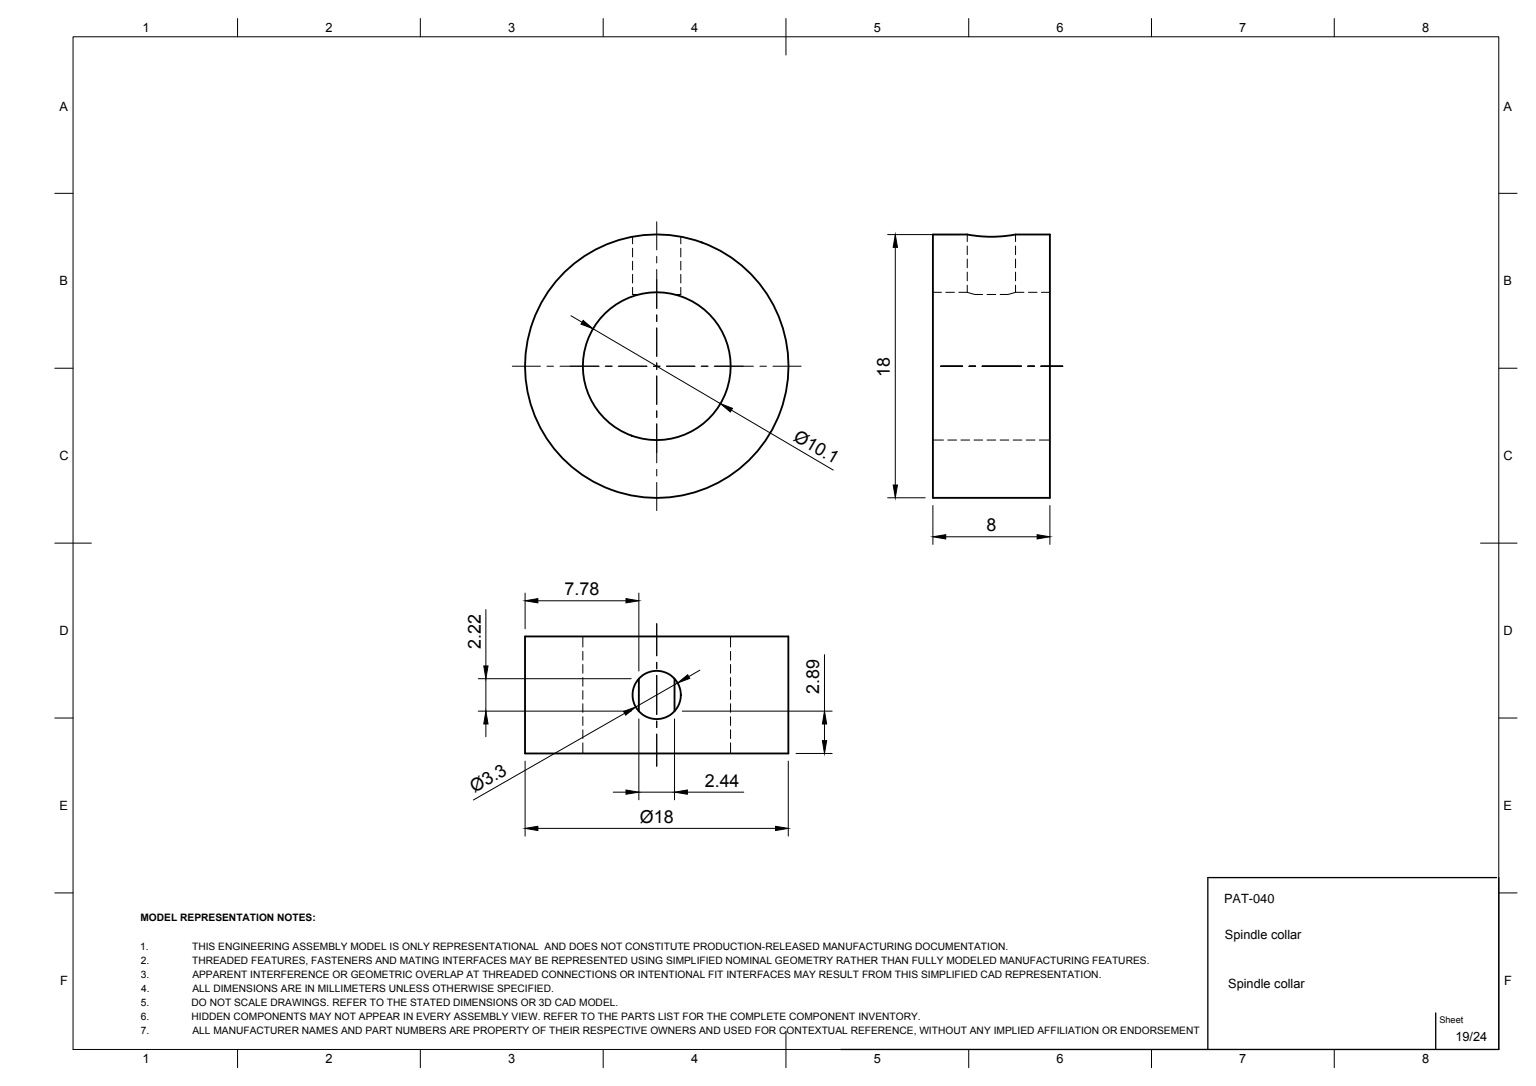
ISO-10303-21;
HEADER;
/* Generated by software containing ST-Developer
 * from STEP Tools, Inc. (www.steptools.com) 
 */

FILE_DESCRIPTION(
/* description */ ('Four-bar tabletop demonstrator'),
/* implementation_level */ '2;1');

FILE_NAME(
/* name */ 'Spindle collar.step',
/* time_stamp */ '2026-10-29T17:05:23-07:00',
/* author */ (''),
/* organization */ (''),
/* preprocessor_version */ 'ST-DEVELOPER v20.2',
/* originating_system */ 'Autodesk Translation Framework v15.17.0.0',
/* authorisation */ '');

FILE_SCHEMA (('AUTOMOTIVE_DESIGN { 1 0 10303 214 3 1 1 }'));
ENDSEC;

DATA;
#10=MECHANICAL_DESIGN_GEOMETRIC_PRESENTATION_REPRESENTATION('',(#358),#6705);
#302=B_SPLINE_CURVE_WITH_KNOTS('',3,(#6493,#6494,#6495,#6496,#6497,#6498,
#6499,#6500,#6501,#6502,#6503,#6504,#6505,#6506),.UNSPECIFIED.,.F.,.F.,
(4,2,2,2,2,2,4),(0.618551524396293,0.626563103102765,0.689203386094988,
0.751843669087211,0.814483952079434,0.877124235071657,0.88513581377813),
 .UNSPECIFIED.);
#303=B_SPLINE_CURVE_WITH_KNOTS('',3,(#6510,#6511,#6512,#6513,#6514,#6515,
#6516,#6517),.UNSPECIFIED.,.F.,.F.,(4,2,2,4),(0.250614556362404,0.313254839354627,
0.37589512234685,0.383906701053323),.UNSPECIFIED.);
#304=B_SPLINE_CURVE_WITH_KNOTS('',3,(#6521,#6522,#6523,#6524,#6525,#6526,
#6527,#6528,#6529,#6530,#6531,#6532,#6533,#6534,#6535,#6536,#6537,#6538,
#6539,#6540,#6541,#6542,#6543,#6544,#6545,#6546),.UNSPECIFIED.,.F.,.F.,
(4,2,2,2,2,2,2,2,2,2,2,2,4),(0.,0.0623062782223143,0.124612556444629,0.186916384615149,
0.249220212785669,0.31152404095619,0.37382786912671,0.436134147349024,0.498440425571339,
0.560746703793653,0.623052982015967,0.685356810186488,0.747660638357008),
 .UNSPECIFIED.);
#305=B_SPLINE_CURVE_WITH_KNOTS('',3,(#6547,#6548,#6549,#6550,#6551,#6552,
#6553,#6554,#6555,#6556),.UNSPECIFIED.,.F.,.F.,(4,2,2,2,4),(0.747660638357008,
0.809964466527528,0.872268294698049,0.934574572920363,0.996880851142677),
 .UNSPECIFIED.);
#306=B_SPLINE_CURVE_WITH_KNOTS('',3,(#6557,#6558,#6559,#6560,#6561,#6562,
#6563,#6564),.UNSPECIFIED.,.F.,.F.,(4,2,2,4),(0.117322411671485,0.125333990377958,
0.187974273370181,0.250614556362404),.UNSPECIFIED.);
#320=SHAPE_REPRESENTATION_RELATIONSHIP('SRR','None',#6830,#335);
#335=ADVANCED_BREP_SHAPE_REPRESENTATION('',(#379),#6703);
#358=STYLED_ITEM('',(#6982),#379);
#379=MANIFOLD_SOLID_BREP('Body1',#3404);
#457=FACE_BOUND('',#1030,.T.);
#458=FACE_BOUND('',#1032,.T.);
#459=FACE_BOUND('',#1034,.T.);
#460=FACE_BOUND('',#1036,.T.);
#549=PLANE('',#4007);
#550=PLANE('',#4011);
#551=PLANE('',#4018);
#552=PLANE('',#4019);
#747=FACE_OUTER_BOUND('',#1026,.T.);
#748=FACE_OUTER_BOUND('',#1027,.T.);
#749=FACE_OUTER_BOUND('',#1028,.T.);
#750=FACE_OUTER_BOUND('',#1029,.T.);
#751=FACE_OUTER_BOUND('',#1031,.T.);
#752=FACE_OUTER_BOUND('',#1033,.T.);
#753=FACE_OUTER_BOUND('',#1035,.T.);
#1026=EDGE_LOOP('',(#3026,#3027));
#1027=EDGE_LOOP('',(#3028,#3029,#3030,#3031,#3032,#3033,#3034,#3035,#3036));
#1028=EDGE_LOOP('',(#3037,#3038));
#1029=EDGE_LOOP('',(#3039,#3040,#3041,#3042));
#1030=EDGE_LOOP('',(#3043,#3044,#3045,#3046,#3047));
#1031=EDGE_LOOP('',(#3048,#3049,#3050,#3051));
#1032=EDGE_LOOP('',(#3052,#3053));
#1033=EDGE_LOOP('',(#3054));
#1034=EDGE_LOOP('',(#3055));
#1035=EDGE_LOOP('',(#3056));
#1036=EDGE_LOOP('',(#3057));
#1194=LINE('',#6489,#1364);
#1195=LINE('',#6519,#1365);
#1196=LINE('',#6566,#1366);
#1197=LINE('',#6571,#1367);
#1198=LINE('',#6577,#1368);
#1364=VECTOR('',#5083,1.);
#1365=VECTOR('',#5090,0.165);
#1366=VECTOR('',#5093,1.);
#1367=VECTOR('',#5098,0.505);
#1368=VECTOR('',#5105,0.9);
#1591=CIRCLE('',#4008,0.165);
#1592=CIRCLE('',#4010,0.165);
#1593=CIRCLE('',#4013,0.505);
#1594=CIRCLE('',#4014,0.505);
#1595=CIRCLE('',#4016,0.9);
#1596=CIRCLE('',#4017,0.9);
#1854=VERTEX_POINT('',#6487);
#1855=VERTEX_POINT('',#6488);
#1856=VERTEX_POINT('',#6492);
#1857=VERTEX_POINT('',#6507);
#1858=VERTEX_POINT('',#6509);
#1859=VERTEX_POINT('',#6518);
#1860=VERTEX_POINT('',#6520);
#1861=VERTEX_POINT('',#6568);
#1862=VERTEX_POINT('',#6570);
#1863=VERTEX_POINT('',#6574);
#1864=VERTEX_POINT('',#6576);
#2249=EDGE_CURVE('',#1854,#1855,#1194,.T.);
#2250=EDGE_CURVE('',#1854,#1855,#1591,.T.);
#2251=EDGE_CURVE('',#1856,#1854,#302,.T.);
#2252=EDGE_CURVE('',#1857,#1856,#1592,.T.);
#2253=EDGE_CURVE('',#1858,#1857,#303,.T.);
#2254=EDGE_CURVE('',#1858,#1859,#1195,.T.);
#2255=EDGE_CURVE('',#1860,#1859,#304,.T.);
#2256=EDGE_CURVE('',#1859,#1860,#305,.T.);
#2257=EDGE_CURVE('',#1855,#1858,#306,.T.);
#2258=EDGE_CURVE('',#1857,#1856,#1196,.T.);
#2259=EDGE_CURVE('',#1861,#1861,#1593,.T.);
#2260=EDGE_CURVE('',#1861,#1862,#1197,.T.);
#2261=EDGE_CURVE('',#1862,#1862,#1594,.T.);
#2262=EDGE_CURVE('',#1863,#1863,#1595,.T.);
#2263=EDGE_CURVE('',#1863,#1864,#1198,.T.);
#2264=EDGE_CURVE('',#1864,#1864,#1596,.T.);
#3026=ORIENTED_EDGE('',*,*,#2249,.F.);
#3027=ORIENTED_EDGE('',*,*,#2250,.T.);
#3028=ORIENTED_EDGE('',*,*,#2251,.F.);
#3029=ORIENTED_EDGE('',*,*,#2252,.F.);
#3030=ORIENTED_EDGE('',*,*,#2253,.F.);
#3031=ORIENTED_EDGE('',*,*,#2254,.T.);
#3032=ORIENTED_EDGE('',*,*,#2255,.F.);
#3033=ORIENTED_EDGE('',*,*,#2256,.F.);
#3034=ORIENTED_EDGE('',*,*,#2254,.F.);
#3035=ORIENTED_EDGE('',*,*,#2257,.F.);
#3036=ORIENTED_EDGE('',*,*,#2250,.F.);
#3037=ORIENTED_EDGE('',*,*,#2258,.F.);
#3038=ORIENTED_EDGE('',*,*,#2252,.T.);
#3039=ORIENTED_EDGE('',*,*,#2259,.F.);
#3040=ORIENTED_EDGE('',*,*,#2260,.T.);
#3041=ORIENTED_EDGE('',*,*,#2261,.T.);
#3042=ORIENTED_EDGE('',*,*,#2260,.F.);
#3043=ORIENTED_EDGE('',*,*,#2257,.T.);
#3044=ORIENTED_EDGE('',*,*,#2253,.T.);
#3045=ORIENTED_EDGE('',*,*,#2258,.T.);
#3046=ORIENTED_EDGE('',*,*,#2251,.T.);
#3047=ORIENTED_EDGE('',*,*,#2249,.T.);
#3048=ORIENTED_EDGE('',*,*,#2262,.F.);
#3049=ORIENTED_EDGE('',*,*,#2263,.T.);
#3050=ORIENTED_EDGE('',*,*,#2264,.T.);
#3051=ORIENTED_EDGE('',*,*,#2263,.F.);
#3052=ORIENTED_EDGE('',*,*,#2255,.T.);
#3053=ORIENTED_EDGE('',*,*,#2256,.T.);
#3054=ORIENTED_EDGE('',*,*,#2262,.T.);
#3055=ORIENTED_EDGE('',*,*,#2259,.T.);
#3056=ORIENTED_EDGE('',*,*,#2264,.F.);
#3057=ORIENTED_EDGE('',*,*,#2261,.F.);
#3174=CYLINDRICAL_SURFACE('',#4009,0.165);
#3175=CYLINDRICAL_SURFACE('',#4012,0.505);
#3176=CYLINDRICAL_SURFACE('',#4015,0.9);
#3363=ADVANCED_FACE('',(#747),#549,.T.);
#3364=ADVANCED_FACE('',(#748),#3174,.F.);
#3365=ADVANCED_FACE('',(#749),#550,.T.);
#3366=ADVANCED_FACE('',(#750,#457),#3175,.F.);
#3367=ADVANCED_FACE('',(#751,#458),#3176,.T.);
#3368=ADVANCED_FACE('',(#752,#459),#551,.T.);
#3369=ADVANCED_FACE('',(#753,#460),#552,.F.);
#3404=CLOSED_SHELL('',(#3363,#3364,#3365,#3366,#3367,#3368,#3369));
#4006=AXIS2_PLACEMENT_3D('',#6485,#5079,#5080);
#4007=AXIS2_PLACEMENT_3D('',#6486,#5081,#5082);
#4008=AXIS2_PLACEMENT_3D('',#6490,#5084,#5085);
#4009=AXIS2_PLACEMENT_3D('',#6491,#5086,#5087);
#4010=AXIS2_PLACEMENT_3D('',#6508,#5088,#5089);
#4011=AXIS2_PLACEMENT_3D('',#6565,#5091,#5092);
#4012=AXIS2_PLACEMENT_3D('',#6567,#5094,#5095);
#4013=AXIS2_PLACEMENT_3D('',#6569,#5096,#5097);
#4014=AXIS2_PLACEMENT_3D('',#6572,#5099,#5100);
#4015=AXIS2_PLACEMENT_3D('',#6573,#5101,#5102);
#4016=AXIS2_PLACEMENT_3D('',#6575,#5103,#5104);
#4017=AXIS2_PLACEMENT_3D('',#6578,#5106,#5107);
#4018=AXIS2_PLACEMENT_3D('',#6579,#5108,#5109);
#4019=AXIS2_PLACEMENT_3D('',#6580,#5110,#5111);
#5079=DIRECTION('axis',(0.,0.,1.));
#5080=DIRECTION('refdir',(1.,0.,0.));
#5081=DIRECTION('center_axis',(1.,0.,0.));
#5082=DIRECTION('ref_axis',(0.,0.,-1.));
#5083=DIRECTION('',(0.,0.,1.));
#5084=DIRECTION('center_axis',(1.,0.,0.));
#5085=DIRECTION('ref_axis',(0.,0.,-1.));
#5086=DIRECTION('center_axis',(1.,0.,0.));
#5087=DIRECTION('ref_axis',(0.,0.,-1.));
#5088=DIRECTION('center_axis',(1.,0.,0.));
#5089=DIRECTION('ref_axis',(0.,0.,-1.));
#5090=DIRECTION('',(1.,0.,0.));
#5091=DIRECTION('center_axis',(1.,0.,0.));
#5092=DIRECTION('ref_axis',(0.,0.,-1.));
#5093=DIRECTION('',(0.,0.,-1.));
#5094=DIRECTION('center_axis',(0.,0.,1.));
#5095=DIRECTION('ref_axis',(1.,0.,0.));
#5096=DIRECTION('center_axis',(0.,0.,-1.));
#5097=DIRECTION('ref_axis',(1.,0.,0.));
#5098=DIRECTION('',(0.,0.,-1.));
#5099=DIRECTION('center_axis',(0.,0.,-1.));
#5100=DIRECTION('ref_axis',(1.,0.,0.));
#5101=DIRECTION('center_axis',(0.,0.,1.));
#5102=DIRECTION('ref_axis',(1.,0.,0.));
#5103=DIRECTION('center_axis',(0.,0.,1.));
#5104=DIRECTION('ref_axis',(1.,0.,0.));
#5105=DIRECTION('',(0.,0.,-1.));
#5106=DIRECTION('center_axis',(0.,0.,1.));
#5107=DIRECTION('ref_axis',(1.,0.,0.));
#5108=DIRECTION('center_axis',(0.,0.,1.));
#5109=DIRECTION('ref_axis',(1.,0.,0.));
#5110=DIRECTION('center_axis',(0.,0.,1.));
#5111=DIRECTION('ref_axis',(1.,0.,0.));
#6485=CARTESIAN_POINT('',(0.,0.,0.));
#6486=CARTESIAN_POINT('Origin',(0.49,0.,1.4));
#6487=CARTESIAN_POINT('',(0.49,0.122167917228706,1.28909463493591));
#6488=CARTESIAN_POINT('',(0.49,0.122167917228706,1.51090536506409));
#6489=CARTESIAN_POINT('',(0.49,0.122167917228706,1.));
#6490=CARTESIAN_POINT('Origin',(0.49,0.,1.4));
#6491=CARTESIAN_POINT('Origin',(0.49,0.,1.4));
#6492=CARTESIAN_POINT('',(0.49,-0.122167917228706,1.28909463493591));
#6493=CARTESIAN_POINT('Ctrl Pts',(0.49,-0.122167917228706,1.28909463493591));
#6494=CARTESIAN_POINT('Ctrl Pts',(0.490448531679987,-0.120368913626296,
1.28711294069536));
#6495=CARTESIAN_POINT('Ctrl Pts',(0.490895245371685,-0.118534896565231,
1.28518965877367));
#6496=CARTESIAN_POINT('Ctrl Pts',(0.494795015531646,-0.102111993019358,
1.2687667552278));
#6497=CARTESIAN_POINT('Ctrl Pts',(0.498442514607594,-0.0836597150224318,
1.25609154388858));
#6498=CARTESIAN_POINT('Ctrl Pts',(0.50357781976106,-0.0430495960471595,
1.23920409039234));
#6499=CARTESIAN_POINT('Ctrl Pts',(0.505,-0.020880094330741,1.235));
#6500=CARTESIAN_POINT('Ctrl Pts',(0.505,0.020880094330741,1.235));
#6501=CARTESIAN_POINT('Ctrl Pts',(0.50357781976106,0.0430495960471595,1.23920409039234));
#6502=CARTESIAN_POINT('Ctrl Pts',(0.498442514607594,0.0836597150224318,
1.25609154388858));
#6503=CARTESIAN_POINT('Ctrl Pts',(0.494795015531646,0.102111993019358,1.2687667552278));
#6504=CARTESIAN_POINT('Ctrl Pts',(0.490895245371684,0.118534896565231,1.28518965877367));
#6505=CARTESIAN_POINT('Ctrl Pts',(0.490448531679987,0.120368913626296,1.28711294069536));
#6506=CARTESIAN_POINT('Ctrl Pts',(0.49,0.122167917228706,1.28909463493591));
#6507=CARTESIAN_POINT('',(0.49,-0.122167917228706,1.51090536506409));
#6508=CARTESIAN_POINT('Origin',(0.49,0.,1.4));
#6509=CARTESIAN_POINT('',(0.505,-1.70422299968729E-17,1.565));
#6510=CARTESIAN_POINT('Ctrl Pts',(0.505,-6.93889390390723E-18,1.565));
#6511=CARTESIAN_POINT('Ctrl Pts',(0.505,-0.020880094330741,1.565));
#6512=CARTESIAN_POINT('Ctrl Pts',(0.50357781976106,-0.0430495960471595,
1.56079590960766));
#6513=CARTESIAN_POINT('Ctrl Pts',(0.498442514607594,-0.0836597150224318,
1.54390845611142));
#6514=CARTESIAN_POINT('Ctrl Pts',(0.494795015531646,-0.102111993019358,
1.5312332447722));
#6515=CARTESIAN_POINT('Ctrl Pts',(0.490895245371684,-0.118534896565231,
1.51481034122633));
#6516=CARTESIAN_POINT('Ctrl Pts',(0.490448531679987,-0.120368913626296,
1.51288705930464));
#6517=CARTESIAN_POINT('Ctrl Pts',(0.49,-0.122167917228706,1.51090536506409));
#6518=CARTESIAN_POINT('',(0.9,-2.02066721859313E-17,1.565));
#6519=CARTESIAN_POINT('',(0.49,-2.02066721859313E-17,1.565));
#6520=CARTESIAN_POINT('',(0.884745726183518,0.165,1.4));
#6521=CARTESIAN_POINT('Ctrl Pts',(0.884745726183518,0.165,1.4));
#6522=CARTESIAN_POINT('Ctrl Pts',(0.884745726183518,0.165,1.37923124059256));
#6523=CARTESIAN_POINT('Ctrl Pts',(0.885552759505264,0.160839719007584,1.35711110492666));
#6524=CARTESIAN_POINT('Ctrl Pts',(0.888448648150043,0.143986470216691,1.31647293736623));
#6525=CARTESIAN_POINT('Ctrl Pts',(0.890493604851638,0.131295993814186,1.29795075602263));
#6526=CARTESIAN_POINT('Ctrl Pts',(0.89431723432394,0.102049819008125,1.26870458121656));
#6527=CARTESIAN_POINT('Ctrl Pts',(0.896347088899543,0.0835273920906824,
1.25601365401642));
#6528=CARTESIAN_POINT('Ctrl Pts',(0.899208271860583,0.0428883760934127,
1.23916007816136));
#6529=CARTESIAN_POINT('Ctrl Pts',(0.9,0.0207679427235068,1.235));
#6530=CARTESIAN_POINT('Ctrl Pts',(0.9,-0.0207679427235068,1.235));
#6531=CARTESIAN_POINT('Ctrl Pts',(0.899208271860583,-0.0428883760934127,
1.23916007816136));
#6532=CARTESIAN_POINT('Ctrl Pts',(0.896347088899543,-0.0835273920906823,
1.25601365401642));
#6533=CARTESIAN_POINT('Ctrl Pts',(0.89431723432394,-0.102049819008125,1.26870458121656));
#6534=CARTESIAN_POINT('Ctrl Pts',(0.890493604851638,-0.131295993814186,
1.29795075602263));
#6535=CARTESIAN_POINT('Ctrl Pts',(0.888448648150043,-0.143986470216691,
1.31647293736623));
#6536=CARTESIAN_POINT('Ctrl Pts',(0.885552759505264,-0.160839719007584,
1.35711110492666));
#6537=CARTESIAN_POINT('Ctrl Pts',(0.884745726183518,-0.165,1.37923124059256));
#6538=CARTESIAN_POINT('Ctrl Pts',(0.884745726183518,-0.165,1.42076875940744));
#6539=CARTESIAN_POINT('Ctrl Pts',(0.885552759505264,-0.160839719007584,
1.44288889507334));
#6540=CARTESIAN_POINT('Ctrl Pts',(0.888448648150043,-0.14398647021669,1.48352706263377));
#6541=CARTESIAN_POINT('Ctrl Pts',(0.890493604851638,-0.131295993814186,
1.50204924397737));
#6542=CARTESIAN_POINT('Ctrl Pts',(0.89431723432394,-0.102049819008125,1.53129541878344));
#6543=CARTESIAN_POINT('Ctrl Pts',(0.896347088899543,-0.0835273920906824,
1.54398634598358));
#6544=CARTESIAN_POINT('Ctrl Pts',(0.899208271860583,-0.0428883760934128,
1.56083992183864));
#6545=CARTESIAN_POINT('Ctrl Pts',(0.9,-0.0207679427235068,1.565));
#6546=CARTESIAN_POINT('Ctrl Pts',(0.9,-6.93889390390723E-18,1.565));
#6547=CARTESIAN_POINT('Ctrl Pts',(0.9,-3.46944695195361E-17,1.565));
#6548=CARTESIAN_POINT('Ctrl Pts',(0.9,0.0207679427235068,1.565));
#6549=CARTESIAN_POINT('Ctrl Pts',(0.899208271860583,0.0428883760934127,
1.56083992183864));
#6550=CARTESIAN_POINT('Ctrl Pts',(0.896347088899543,0.0835273920906824,
1.54398634598358));
#6551=CARTESIAN_POINT('Ctrl Pts',(0.89431723432394,0.102049819008125,1.53129541878344));
#6552=CARTESIAN_POINT('Ctrl Pts',(0.890493604851638,0.131295993814186,1.50204924397737));
#6553=CARTESIAN_POINT('Ctrl Pts',(0.888448648150043,0.143986470216691,1.48352706263377));
#6554=CARTESIAN_POINT('Ctrl Pts',(0.885552759505264,0.160839719007584,1.44288889507334));
#6555=CARTESIAN_POINT('Ctrl Pts',(0.884745726183518,0.165,1.42076875940744));
#6556=CARTESIAN_POINT('Ctrl Pts',(0.884745726183518,0.165,1.4));
#6557=CARTESIAN_POINT('Ctrl Pts',(0.49,0.122167917228706,1.51090536506409));
#6558=CARTESIAN_POINT('Ctrl Pts',(0.490448531679987,0.120368913626296,1.51288705930464));
#6559=CARTESIAN_POINT('Ctrl Pts',(0.490895245371685,0.118534896565231,1.51481034122633));
#6560=CARTESIAN_POINT('Ctrl Pts',(0.494795015531646,0.102111993019358,1.5312332447722));
#6561=CARTESIAN_POINT('Ctrl Pts',(0.498442514607594,0.0836597150224318,
1.54390845611142));
#6562=CARTESIAN_POINT('Ctrl Pts',(0.50357781976106,0.0430495960471594,1.56079590960766));
#6563=CARTESIAN_POINT('Ctrl Pts',(0.505,0.020880094330741,1.565));
#6564=CARTESIAN_POINT('Ctrl Pts',(0.505,0.,1.565));
#6565=CARTESIAN_POINT('Origin',(0.49,0.,1.4));
#6566=CARTESIAN_POINT('',(0.49,-0.122167917228706,1.));
#6567=CARTESIAN_POINT('Origin',(0.,0.,1.));
#6568=CARTESIAN_POINT('',(-0.505,-6.18446633569413E-17,1.8));
#6569=CARTESIAN_POINT('Origin',(0.,0.,1.8));
#6570=CARTESIAN_POINT('',(-0.505,-6.18446633569413E-17,1.));
#6571=CARTESIAN_POINT('',(-0.505,-6.18446633569413E-17,1.));
#6572=CARTESIAN_POINT('Origin',(0.,0.,1.));
#6573=CARTESIAN_POINT('Origin',(0.,0.,1.));
#6574=CARTESIAN_POINT('',(-0.9,-1.10218211923262E-16,1.8));
#6575=CARTESIAN_POINT('Origin',(0.,0.,1.8));
#6576=CARTESIAN_POINT('',(-0.9,-1.10218211923262E-16,1.));
#6577=CARTESIAN_POINT('',(-0.9,-1.10218211923262E-16,1.));
#6578=CARTESIAN_POINT('Origin',(0.,0.,1.));
#6579=CARTESIAN_POINT('Origin',(0.,0.,1.8));
#6580=CARTESIAN_POINT('Origin',(0.,0.,1.));
#6681=UNCERTAINTY_MEASURE_WITH_UNIT(LENGTH_MEASURE(0.001),#6706,
'DISTANCE_ACCURACY_VALUE',
'Maximum model space distance between geometric entities at asserted c
onnectivities');
#6683=UNCERTAINTY_MEASURE_WITH_UNIT(LENGTH_MEASURE(0.001),#6706,
'DISTANCE_ACCURACY_VALUE',
'Maximum model space distance between geometric entities at asserted c
onnectivities');
#6703=(
GEOMETRIC_REPRESENTATION_CONTEXT(3)
GLOBAL_UNCERTAINTY_ASSIGNED_CONTEXT((#6681))
GLOBAL_UNIT_ASSIGNED_CONTEXT((#6706,#6708,#6709))
REPRESENTATION_CONTEXT('','3D')
);
#6705=(
GEOMETRIC_REPRESENTATION_CONTEXT(3)
GLOBAL_UNCERTAINTY_ASSIGNED_CONTEXT((#6683))
GLOBAL_UNIT_ASSIGNED_CONTEXT((#6706,#6708,#6709))
REPRESENTATION_CONTEXT('','3D')
);
#6706=(
LENGTH_UNIT()
NAMED_UNIT(*)
SI_UNIT(.CENTI.,.METRE.)
);
#6708=(
NAMED_UNIT(*)
PLANE_ANGLE_UNIT()
SI_UNIT($,.RADIAN.)
);
#6709=(
NAMED_UNIT(*)
SI_UNIT($,.STERADIAN.)
SOLID_ANGLE_UNIT()
);
#6729=SHAPE_DEFINITION_REPRESENTATION(#6778,#6830);
#6778=PRODUCT_DEFINITION_SHAPE('',$,#6852);
#6830=SHAPE_REPRESENTATION('',(#4006),#6703);
#6832=PRODUCT_DEFINITION_CONTEXT('part definition',#6897,'design');
#6852=PRODUCT_DEFINITION('Spindle collar','Spindle collar',#6873,#6832);
#6873=PRODUCT_DEFINITION_FORMATION('',$,#6918);
#6897=APPLICATION_CONTEXT(
'Core Data for Automotive Mechanical Design Process');
#6898=PRODUCT_CONTEXT('part definition',#6897,'mechanical');
#6918=PRODUCT('Spindle collar','Spindle collar','Spindle collar',(#6898));
#6976=COLOUR_RGB('Sky Blue',0.24,0.69,0.87);
#6977=FILL_AREA_STYLE_COLOUR('',#6976);
#6978=FILL_AREA_STYLE('',(#6977));
#6979=SURFACE_STYLE_FILL_AREA(#6978);
#6980=SURFACE_SIDE_STYLE('',(#6979));
#6981=SURFACE_STYLE_USAGE(.BOTH.,#6980);
#6982=PRESENTATION_STYLE_ASSIGNMENT((#6981));
ENDSEC;
END-ISO-10303-21;
